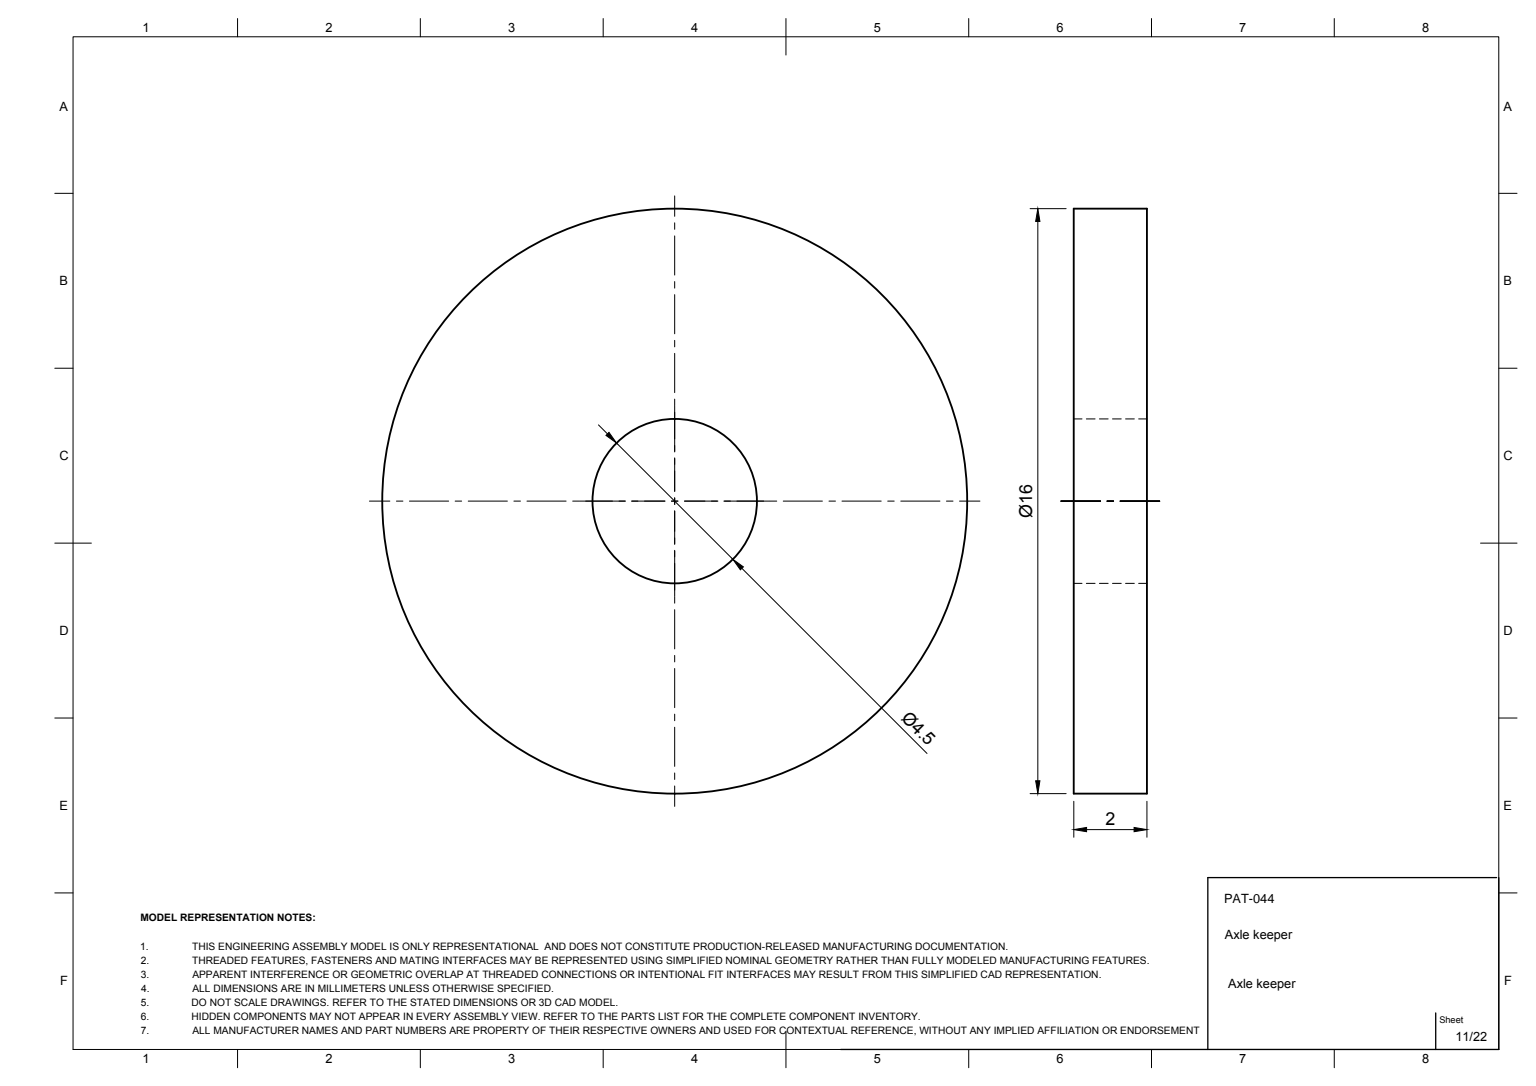
ISO-10303-21;
HEADER;
/* Generated by software containing ST-Developer
 * from STEP Tools, Inc. (www.steptools.com) 
 */

FILE_DESCRIPTION(
/* description */ ('Four-wheel beam trolley'),
/* implementation_level */ '2;1');

FILE_NAME(
/* name */ 'Axle keeper.step',
/* time_stamp */ '2026-10-29T16:22:06-07:00',
/* author */ (''),
/* organization */ (''),
/* preprocessor_version */ 'ST-DEVELOPER v20.2',
/* originating_system */ 'Autodesk Translation Framework v15.17.0.0',
/* authorisation */ '');

FILE_SCHEMA (('AUTOMOTIVE_DESIGN { 1 0 10303 214 3 1 1 }'));
ENDSEC;

DATA;
#10=MECHANICAL_DESIGN_GEOMETRIC_PRESENTATION_REPRESENTATION('',(#286),#4777);
#252=SHAPE_REPRESENTATION_RELATIONSHIP('SRR','None',#4881,#269);
#269=ADVANCED_BREP_SHAPE_REPRESENTATION('',(#309),#4766);
#286=STYLED_ITEM('',(#5056),#309);
#309=MANIFOLD_SOLID_BREP('Body1',#2374);
#347=FACE_BOUND('',#682,.T.);
#348=FACE_BOUND('',#684,.T.);
#407=PLANE('',#2709);
#408=PLANE('',#2710);
#509=FACE_OUTER_BOUND('',#679,.T.);
#510=FACE_OUTER_BOUND('',#680,.T.);
#511=FACE_OUTER_BOUND('',#681,.T.);
#512=FACE_OUTER_BOUND('',#683,.T.);
#679=EDGE_LOOP('',(#1869,#1870,#1871,#1872));
#680=EDGE_LOOP('',(#1873,#1874,#1875,#1876));
#681=EDGE_LOOP('',(#1877));
#682=EDGE_LOOP('',(#1878));
#683=EDGE_LOOP('',(#1879));
#684=EDGE_LOOP('',(#1880));
#853=LINE('',#4045,#976);
#854=LINE('',#4051,#977);
#976=VECTOR('',#3260,0.225);
#977=VECTOR('',#3267,0.8);
#1069=CIRCLE('',#2704,0.225);
#1070=CIRCLE('',#2705,0.225);
#1071=CIRCLE('',#2707,0.8);
#1072=CIRCLE('',#2708,0.8);
#1241=VERTEX_POINT('',#4042);
#1242=VERTEX_POINT('',#4044);
#1243=VERTEX_POINT('',#4048);
#1244=VERTEX_POINT('',#4050);
#1472=EDGE_CURVE('',#1241,#1241,#1069,.T.);
#1473=EDGE_CURVE('',#1241,#1242,#853,.T.);
#1474=EDGE_CURVE('',#1242,#1242,#1070,.T.);
#1475=EDGE_CURVE('',#1243,#1243,#1071,.T.);
#1476=EDGE_CURVE('',#1243,#1244,#854,.T.);
#1477=EDGE_CURVE('',#1244,#1244,#1072,.T.);
#1869=ORIENTED_EDGE('',*,*,#1472,.F.);
#1870=ORIENTED_EDGE('',*,*,#1473,.T.);
#1871=ORIENTED_EDGE('',*,*,#1474,.T.);
#1872=ORIENTED_EDGE('',*,*,#1473,.F.);
#1873=ORIENTED_EDGE('',*,*,#1475,.F.);
#1874=ORIENTED_EDGE('',*,*,#1476,.T.);
#1875=ORIENTED_EDGE('',*,*,#1477,.T.);
#1876=ORIENTED_EDGE('',*,*,#1476,.F.);
#1877=ORIENTED_EDGE('',*,*,#1475,.T.);
#1878=ORIENTED_EDGE('',*,*,#1472,.T.);
#1879=ORIENTED_EDGE('',*,*,#1477,.F.);
#1880=ORIENTED_EDGE('',*,*,#1474,.F.);
#2196=CYLINDRICAL_SURFACE('',#2703,0.225);
#2197=CYLINDRICAL_SURFACE('',#2706,0.8);
#2285=ADVANCED_FACE('',(#509),#2196,.F.);
#2286=ADVANCED_FACE('',(#510),#2197,.T.);
#2287=ADVANCED_FACE('',(#511,#347),#407,.T.);
#2288=ADVANCED_FACE('',(#512,#348),#408,.F.);
#2374=CLOSED_SHELL('',(#2285,#2286,#2287,#2288));
#2702=AXIS2_PLACEMENT_3D('',#4040,#3254,#3255);
#2703=AXIS2_PLACEMENT_3D('',#4041,#3256,#3257);
#2704=AXIS2_PLACEMENT_3D('',#4043,#3258,#3259);
#2705=AXIS2_PLACEMENT_3D('',#4046,#3261,#3262);
#2706=AXIS2_PLACEMENT_3D('',#4047,#3263,#3264);
#2707=AXIS2_PLACEMENT_3D('',#4049,#3265,#3266);
#2708=AXIS2_PLACEMENT_3D('',#4052,#3268,#3269);
#2709=AXIS2_PLACEMENT_3D('',#4053,#3270,#3271);
#2710=AXIS2_PLACEMENT_3D('',#4054,#3272,#3273);
#3254=DIRECTION('axis',(0.,0.,1.));
#3255=DIRECTION('refdir',(1.,0.,0.));
#3256=DIRECTION('center_axis',(0.,1.,0.));
#3257=DIRECTION('ref_axis',(1.,0.,0.));
#3258=DIRECTION('center_axis',(0.,-1.,0.));
#3259=DIRECTION('ref_axis',(1.,0.,0.));
#3260=DIRECTION('',(0.,-1.,0.));
#3261=DIRECTION('center_axis',(0.,-1.,0.));
#3262=DIRECTION('ref_axis',(1.,0.,0.));
#3263=DIRECTION('center_axis',(0.,1.,0.));
#3264=DIRECTION('ref_axis',(1.,0.,0.));
#3265=DIRECTION('center_axis',(0.,1.,0.));
#3266=DIRECTION('ref_axis',(1.,0.,0.));
#3267=DIRECTION('',(0.,-1.,0.));
#3268=DIRECTION('center_axis',(0.,1.,0.));
#3269=DIRECTION('ref_axis',(1.,0.,0.));
#3270=DIRECTION('center_axis',(0.,1.,0.));
#3271=DIRECTION('ref_axis',(1.,0.,0.));
#3272=DIRECTION('center_axis',(0.,1.,0.));
#3273=DIRECTION('ref_axis',(1.,0.,0.));
#4040=CARTESIAN_POINT('',(0.,0.,0.));
#4041=CARTESIAN_POINT('Origin',(0.,2.2,4.));
#4042=CARTESIAN_POINT('',(-0.225,2.4,4.));
#4043=CARTESIAN_POINT('Origin',(0.,2.4,4.));
#4044=CARTESIAN_POINT('',(-0.225,2.2,4.));
#4045=CARTESIAN_POINT('',(-0.225,2.2,4.));
#4046=CARTESIAN_POINT('Origin',(0.,2.2,4.));
#4047=CARTESIAN_POINT('Origin',(0.,2.2,4.));
#4048=CARTESIAN_POINT('',(-0.8,2.4,4.));
#4049=CARTESIAN_POINT('Origin',(0.,2.4,4.));
#4050=CARTESIAN_POINT('',(-0.8,2.2,4.));
#4051=CARTESIAN_POINT('',(-0.8,2.2,4.));
#4052=CARTESIAN_POINT('Origin',(0.,2.2,4.));
#4053=CARTESIAN_POINT('Origin',(0.,2.4,4.));
#4054=CARTESIAN_POINT('Origin',(0.,2.2,4.));
#4744=UNCERTAINTY_MEASURE_WITH_UNIT(LENGTH_MEASURE(0.001),#4778,
'DISTANCE_ACCURACY_VALUE',
'Maximum model space distance between geometric entities at asserted c
onnectivities');
#4755=UNCERTAINTY_MEASURE_WITH_UNIT(LENGTH_MEASURE(0.001),#4778,
'DISTANCE_ACCURACY_VALUE',
'Maximum model space distance between geometric entities at asserted c
onnectivities');
#4766=(
GEOMETRIC_REPRESENTATION_CONTEXT(3)
GLOBAL_UNCERTAINTY_ASSIGNED_CONTEXT((#4744))
GLOBAL_UNIT_ASSIGNED_CONTEXT((#4778,#4780,#4781))
REPRESENTATION_CONTEXT('','3D')
);
#4777=(
GEOMETRIC_REPRESENTATION_CONTEXT(3)
GLOBAL_UNCERTAINTY_ASSIGNED_CONTEXT((#4755))
GLOBAL_UNIT_ASSIGNED_CONTEXT((#4778,#4780,#4781))
REPRESENTATION_CONTEXT('','3D')
);
#4778=(
LENGTH_UNIT()
NAMED_UNIT(*)
SI_UNIT(.CENTI.,.METRE.)
);
#4780=(
NAMED_UNIT(*)
PLANE_ANGLE_UNIT()
SI_UNIT($,.RADIAN.)
);
#4781=(
NAMED_UNIT(*)
SI_UNIT($,.STERADIAN.)
SOLID_ANGLE_UNIT()
);
#4792=SHAPE_DEFINITION_REPRESENTATION(#4813,#4881);
#4813=PRODUCT_DEFINITION_SHAPE('',$,#4903);
#4881=SHAPE_REPRESENTATION('',(#2702),#4766);
#4892=PRODUCT_DEFINITION_CONTEXT('part definition',#4957,'design');
#4903=PRODUCT_DEFINITION('Axle keeper','Axle keeper',#4924,#4892);
#4924=PRODUCT_DEFINITION_FORMATION('',$,#4969);
#4957=APPLICATION_CONTEXT(
'Core Data for Automotive Mechanical Design Process');
#4958=PRODUCT_CONTEXT('part definition',#4957,'mechanical');
#4969=PRODUCT('Axle keeper','Axle keeper','Axle keeper',(#4958));
#5050=COLOUR_RGB('Grey',0.48,0.52,0.57);
#5051=FILL_AREA_STYLE_COLOUR('',#5050);
#5052=FILL_AREA_STYLE('',(#5051));
#5053=SURFACE_STYLE_FILL_AREA(#5052);
#5054=SURFACE_SIDE_STYLE('',(#5053));
#5055=SURFACE_STYLE_USAGE(.BOTH.,#5054);
#5056=PRESENTATION_STYLE_ASSIGNMENT((#5055));
ENDSEC;
END-ISO-10303-21;
